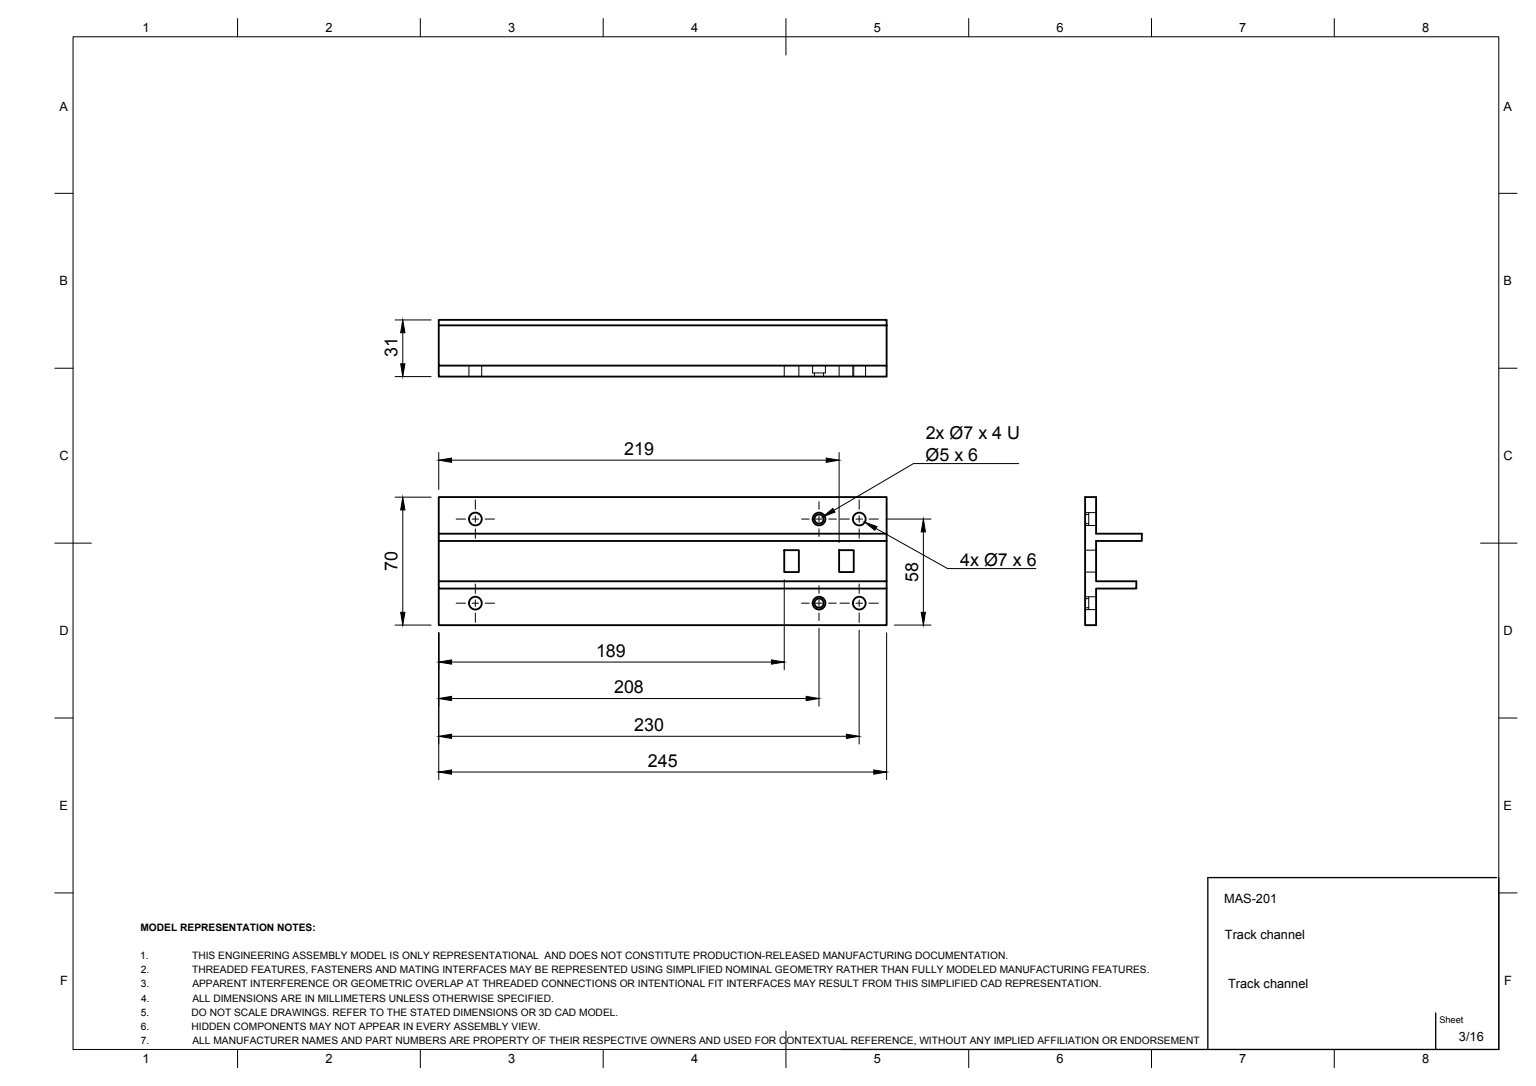
ISO-10303-21;
HEADER;
/* Generated by software containing ST-Developer
 * from STEP Tools, Inc. (www.steptools.com) 
 */

FILE_DESCRIPTION(
/* description */ ('Independent manual two-gate roller-track escapement for nominal30mm d
iameter20mm wide feed rollers. Opposed gates are driven by native capt
ured pin-slot loops with positive curved-slot travel stops at\X\B116de
g. Repeated gate/pin/washer/clip instances, adapted native common bear
ing families, full retaining lips and rotating polymer grip. External 
workpieces, gravity feeder/incline and mount anchors outside assembly.
 No powered-feed compatibility, impact, capacity, safety, force, wear 
or life rating.'),
/* implementation_level */ '2;1');

FILE_NAME(
/* name */ 'Track channel.step',
/* time_stamp */ '2026-11-08T18:43:23-08:00',
/* author */ (''),
/* organization */ (''),
/* preprocessor_version */ 'ST-DEVELOPER v20.2',
/* originating_system */ 'Autodesk Translation Framework v15.17.0.0',
/* authorisation */ '');

FILE_SCHEMA (('AUTOMOTIVE_DESIGN { 1 0 10303 214 3 1 1 }'));
ENDSEC;

DATA;
#10=MECHANICAL_DESIGN_GEOMETRIC_PRESENTATION_REPRESENTATION('',(#455),#19863);
#417=SHAPE_REPRESENTATION_RELATIONSHIP('SRR','None',#19935,#436);
#436=ADVANCED_BREP_SHAPE_REPRESENTATION('',(#474),#19844);
#455=STYLED_ITEM('',(#20039),#474);
#474=MANIFOLD_SOLID_BREP('Body1',#6424);
#493=LINE('',#8742,#958);
#494=LINE('',#8745,#959);
#495=LINE('',#8755,#960);
#496=LINE('',#8758,#961);
#497=LINE('',#8764,#962);
#498=LINE('',#8770,#963);
#499=LINE('',#8776,#964);
#500=LINE('',#8782,#965);
#501=LINE('',#8787,#966);
#502=LINE('',#8789,#967);
#503=LINE('',#8791,#968);
#504=LINE('',#8792,#969);
#505=LINE('',#8795,#970);
#506=LINE('',#8797,#971);
#507=LINE('',#8798,#972);
#508=LINE('',#8801,#973);
#509=LINE('',#8803,#974);
#510=LINE('',#8804,#975);
#511=LINE('',#8806,#976);
#512=LINE('',#8807,#977);
#513=LINE('',#8811,#978);
#514=LINE('',#8813,#979);
#515=LINE('',#8815,#980);
#516=LINE('',#8816,#981);
#517=LINE('',#8819,#982);
#518=LINE('',#8821,#983);
#519=LINE('',#8822,#984);
#520=LINE('',#8825,#985);
#521=LINE('',#8827,#986);
#522=LINE('',#8828,#987);
#523=LINE('',#8830,#988);
#524=LINE('',#8831,#989);
#525=LINE('',#8835,#990);
#526=LINE('',#8837,#991);
#527=LINE('',#8839,#992);
#528=LINE('',#8840,#993);
#529=LINE('',#8844,#994);
#530=LINE('',#8846,#995);
#531=LINE('',#8848,#996);
#532=LINE('',#8849,#997);
#533=LINE('',#8851,#998);
#534=LINE('',#8852,#999);
#535=LINE('',#8855,#1000);
#536=LINE('',#8857,#1001);
#537=LINE('',#8858,#1002);
#538=LINE('',#8861,#1003);
#539=LINE('',#8863,#1004);
#540=LINE('',#8864,#1005);
#541=LINE('',#8867,#1006);
#542=LINE('',#8869,#1007);
#543=LINE('',#8870,#1008);
#544=LINE('',#8874,#1009);
#545=LINE('',#8876,#1010);
#546=LINE('',#8878,#1011);
#547=LINE('',#8879,#1012);
#548=LINE('',#8881,#1013);
#549=LINE('',#8882,#1014);
#550=LINE('',#8885,#1015);
#551=LINE('',#8887,#1016);
#552=LINE('',#8888,#1017);
#553=LINE('',#8892,#1018);
#554=LINE('',#8893,#1019);
#555=LINE('',#8894,#1020);
#556=LINE('',#8897,#1021);
#557=LINE('',#8898,#1022);
#558=LINE('',#8901,#1023);
#559=LINE('',#8902,#1024);
#560=LINE('',#8904,#1025);
#958=VECTOR('',#7205,3.5);
#959=VECTOR('',#7208,2.5);
#960=VECTOR('',#7221,3.5);
#961=VECTOR('',#7224,2.5);
#962=VECTOR('',#7231,3.5);
#963=VECTOR('',#7238,3.5);
#964=VECTOR('',#7245,3.5);
#965=VECTOR('',#7252,3.5);
#966=VECTOR('',#7257,10.);
#967=VECTOR('',#7258,10.);
#968=VECTOR('',#7259,10.);
#969=VECTOR('',#7260,10.);
#970=VECTOR('',#7263,10.);
#971=VECTOR('',#7264,10.);
#972=VECTOR('',#7265,10.);
#973=VECTOR('',#7268,10.);
#974=VECTOR('',#7269,10.);
#975=VECTOR('',#7270,10.);
#976=VECTOR('',#7273,10.);
#977=VECTOR('',#7274,10.);
#978=VECTOR('',#7277,10.);
#979=VECTOR('',#7278,10.);
#980=VECTOR('',#7279,10.);
#981=VECTOR('',#7280,10.);
#982=VECTOR('',#7283,10.);
#983=VECTOR('',#7284,10.);
#984=VECTOR('',#7285,10.);
#985=VECTOR('',#7288,10.);
#986=VECTOR('',#7289,10.);
#987=VECTOR('',#7290,10.);
#988=VECTOR('',#7293,10.);
#989=VECTOR('',#7294,10.);
#990=VECTOR('',#7297,10.);
#991=VECTOR('',#7298,10.);
#992=VECTOR('',#7299,10.);
#993=VECTOR('',#7300,10.);
#994=VECTOR('',#7303,10.);
#995=VECTOR('',#7304,10.);
#996=VECTOR('',#7305,10.);
#997=VECTOR('',#7306,10.);
#998=VECTOR('',#7309,10.);
#999=VECTOR('',#7310,10.);
#1000=VECTOR('',#7313,10.);
#1001=VECTOR('',#7314,10.);
#1002=VECTOR('',#7315,10.);
#1003=VECTOR('',#7318,10.);
#1004=VECTOR('',#7319,10.);
#1005=VECTOR('',#7320,10.);
#1006=VECTOR('',#7323,10.);
#1007=VECTOR('',#7324,10.);
#1008=VECTOR('',#7325,10.);
#1009=VECTOR('',#7328,10.);
#1010=VECTOR('',#7329,10.);
#1011=VECTOR('',#7330,10.);
#1012=VECTOR('',#7331,10.);
#1013=VECTOR('',#7334,10.);
#1014=VECTOR('',#7335,10.);
#1015=VECTOR('',#7338,10.);
#1016=VECTOR('',#7339,10.);
#1017=VECTOR('',#7340,10.);
#1018=VECTOR('',#7343,10.);
#1019=VECTOR('',#7344,10.);
#1020=VECTOR('',#7345,10.);
#1021=VECTOR('',#7348,10.);
#1022=VECTOR('',#7349,10.);
#1023=VECTOR('',#7352,10.);
#1024=VECTOR('',#7353,10.);
#1025=VECTOR('',#7356,10.);
#1423=CYLINDRICAL_SURFACE('',#6658,3.5);
#1424=CYLINDRICAL_SURFACE('',#6660,2.5);
#1425=CYLINDRICAL_SURFACE('',#6665,3.5);
#1426=CYLINDRICAL_SURFACE('',#6667,2.5);
#1427=CYLINDRICAL_SURFACE('',#6669,3.5);
#1428=CYLINDRICAL_SURFACE('',#6672,3.5);
#1429=CYLINDRICAL_SURFACE('',#6675,3.5);
#1430=CYLINDRICAL_SURFACE('',#6678,3.5);
#1616=FACE_BOUND('',#2046,.T.);
#1617=FACE_BOUND('',#2050,.T.);
#1618=FACE_BOUND('',#2069,.T.);
#1619=FACE_BOUND('',#2070,.T.);
#1620=FACE_BOUND('',#2071,.T.);
#1621=FACE_BOUND('',#2073,.T.);
#1622=FACE_BOUND('',#2074,.T.);
#1623=FACE_BOUND('',#2079,.T.);
#1624=FACE_BOUND('',#2080,.T.);
#1625=FACE_BOUND('',#2081,.T.);
#1626=FACE_BOUND('',#2087,.T.);
#1627=FACE_BOUND('',#2088,.T.);
#1628=FACE_BOUND('',#2089,.T.);
#1629=FACE_BOUND('',#2090,.T.);
#1630=FACE_BOUND('',#2091,.T.);
#1631=FACE_BOUND('',#2092,.T.);
#1632=FACE_BOUND('',#2093,.T.);
#1633=FACE_BOUND('',#2094,.T.);
#1687=FACE_OUTER_BOUND('',#2045,.T.);
#1688=FACE_OUTER_BOUND('',#2047,.T.);
#1689=FACE_OUTER_BOUND('',#2048,.T.);
#1690=FACE_OUTER_BOUND('',#2049,.T.);
#1691=FACE_OUTER_BOUND('',#2051,.T.);
#1692=FACE_OUTER_BOUND('',#2052,.T.);
#1693=FACE_OUTER_BOUND('',#2053,.T.);
#1694=FACE_OUTER_BOUND('',#2054,.T.);
#1695=FACE_OUTER_BOUND('',#2055,.T.);
#1696=FACE_OUTER_BOUND('',#2056,.T.);
#1697=FACE_OUTER_BOUND('',#2057,.T.);
#1698=FACE_OUTER_BOUND('',#2058,.T.);
#1699=FACE_OUTER_BOUND('',#2059,.T.);
#1700=FACE_OUTER_BOUND('',#2060,.T.);
#1701=FACE_OUTER_BOUND('',#2061,.T.);
#1702=FACE_OUTER_BOUND('',#2062,.T.);
#1703=FACE_OUTER_BOUND('',#2063,.T.);
#1704=FACE_OUTER_BOUND('',#2064,.T.);
#1705=FACE_OUTER_BOUND('',#2065,.T.);
#1706=FACE_OUTER_BOUND('',#2066,.T.);
#1707=FACE_OUTER_BOUND('',#2067,.T.);
#1708=FACE_OUTER_BOUND('',#2068,.T.);
#1709=FACE_OUTER_BOUND('',#2072,.T.);
#1710=FACE_OUTER_BOUND('',#2075,.T.);
#1711=FACE_OUTER_BOUND('',#2076,.T.);
#1712=FACE_OUTER_BOUND('',#2077,.T.);
#1713=FACE_OUTER_BOUND('',#2078,.T.);
#1714=FACE_OUTER_BOUND('',#2082,.T.);
#1715=FACE_OUTER_BOUND('',#2083,.T.);
#1716=FACE_OUTER_BOUND('',#2084,.T.);
#1717=FACE_OUTER_BOUND('',#2085,.T.);
#1718=FACE_OUTER_BOUND('',#2086,.T.);
#2045=EDGE_LOOP('',(#4115));
#2046=EDGE_LOOP('',(#4116));
#2047=EDGE_LOOP('',(#4117,#4118,#4119,#4120));
#2048=EDGE_LOOP('',(#4121,#4122,#4123,#4124));
#2049=EDGE_LOOP('',(#4125));
#2050=EDGE_LOOP('',(#4126));
#2051=EDGE_LOOP('',(#4127,#4128,#4129,#4130));
#2052=EDGE_LOOP('',(#4131,#4132,#4133,#4134));
#2053=EDGE_LOOP('',(#4135,#4136,#4137,#4138));
#2054=EDGE_LOOP('',(#4139,#4140,#4141,#4142));
#2055=EDGE_LOOP('',(#4143,#4144,#4145,#4146));
#2056=EDGE_LOOP('',(#4147,#4148,#4149,#4150));
#2057=EDGE_LOOP('',(#4151,#4152,#4153,#4154));
#2058=EDGE_LOOP('',(#4155,#4156,#4157,#4158));
#2059=EDGE_LOOP('',(#4159,#4160,#4161,#4162));
#2060=EDGE_LOOP('',(#4163,#4164,#4165,#4166));
#2061=EDGE_LOOP('',(#4167,#4168,#4169,#4170));
#2062=EDGE_LOOP('',(#4171,#4172,#4173,#4174));
#2063=EDGE_LOOP('',(#4175,#4176,#4177,#4178));
#2064=EDGE_LOOP('',(#4179,#4180,#4181,#4182));
#2065=EDGE_LOOP('',(#4183,#4184,#4185,#4186));
#2066=EDGE_LOOP('',(#4187,#4188,#4189,#4190));
#2067=EDGE_LOOP('',(#4191,#4192,#4193,#4194));
#2068=EDGE_LOOP('',(#4195,#4196,#4197,#4198));
#2069=EDGE_LOOP('',(#4199));
#2070=EDGE_LOOP('',(#4200));
#2071=EDGE_LOOP('',(#4201));
#2072=EDGE_LOOP('',(#4202,#4203,#4204,#4205));
#2073=EDGE_LOOP('',(#4206,#4207,#4208,#4209));
#2074=EDGE_LOOP('',(#4210,#4211,#4212,#4213));
#2075=EDGE_LOOP('',(#4214,#4215,#4216,#4217));
#2076=EDGE_LOOP('',(#4218,#4219,#4220,#4221));
#2077=EDGE_LOOP('',(#4222,#4223,#4224,#4225));
#2078=EDGE_LOOP('',(#4226,#4227,#4228,#4229));
#2079=EDGE_LOOP('',(#4230));
#2080=EDGE_LOOP('',(#4231));
#2081=EDGE_LOOP('',(#4232));
#2082=EDGE_LOOP('',(#4233,#4234,#4235,#4236));
#2083=EDGE_LOOP('',(#4237,#4238,#4239,#4240,#4241,#4242,#4243,#4244,#4245,
#4246,#4247,#4248));
#2084=EDGE_LOOP('',(#4249,#4250,#4251,#4252));
#2085=EDGE_LOOP('',(#4253,#4254,#4255,#4256,#4257,#4258,#4259,#4260,#4261,
#4262,#4263,#4264));
#2086=EDGE_LOOP('',(#4265,#4266,#4267,#4268));
#2087=EDGE_LOOP('',(#4269));
#2088=EDGE_LOOP('',(#4270));
#2089=EDGE_LOOP('',(#4271));
#2090=EDGE_LOOP('',(#4272));
#2091=EDGE_LOOP('',(#4273,#4274,#4275,#4276));
#2092=EDGE_LOOP('',(#4277,#4278,#4279,#4280));
#2093=EDGE_LOOP('',(#4281));
#2094=EDGE_LOOP('',(#4282));
#2474=CIRCLE('',#6656,3.5);
#2475=CIRCLE('',#6657,2.5);
#2476=CIRCLE('',#6659,3.5);
#2477=CIRCLE('',#6661,2.5);
#2478=CIRCLE('',#6663,3.5);
#2479=CIRCLE('',#6664,2.5);
#2480=CIRCLE('',#6666,3.5);
#2481=CIRCLE('',#6668,2.5);
#2482=CIRCLE('',#6670,3.5);
#2483=CIRCLE('',#6671,3.5);
#2484=CIRCLE('',#6673,3.5);
#2485=CIRCLE('',#6674,3.5);
#2486=CIRCLE('',#6676,3.5);
#2487=CIRCLE('',#6677,3.5);
#2488=CIRCLE('',#6679,3.5);
#2489=CIRCLE('',#6680,3.5);
#2618=VERTEX_POINT('',#8735);
#2619=VERTEX_POINT('',#8737);
#2620=VERTEX_POINT('',#8740);
#2621=VERTEX_POINT('',#8744);
#2622=VERTEX_POINT('',#8748);
#2623=VERTEX_POINT('',#8750);
#2624=VERTEX_POINT('',#8753);
#2625=VERTEX_POINT('',#8757);
#2626=VERTEX_POINT('',#8761);
#2627=VERTEX_POINT('',#8763);
#2628=VERTEX_POINT('',#8767);
#2629=VERTEX_POINT('',#8769);
#2630=VERTEX_POINT('',#8773);
#2631=VERTEX_POINT('',#8775);
#2632=VERTEX_POINT('',#8779);
#2633=VERTEX_POINT('',#8781);
#2634=VERTEX_POINT('',#8785);
#2635=VERTEX_POINT('',#8786);
#2636=VERTEX_POINT('',#8788);
#2637=VERTEX_POINT('',#8790);
#2638=VERTEX_POINT('',#8794);
#2639=VERTEX_POINT('',#8796);
#2640=VERTEX_POINT('',#8800);
#2641=VERTEX_POINT('',#8802);
#2642=VERTEX_POINT('',#8809);
#2643=VERTEX_POINT('',#8810);
#2644=VERTEX_POINT('',#8812);
#2645=VERTEX_POINT('',#8814);
#2646=VERTEX_POINT('',#8818);
#2647=VERTEX_POINT('',#8820);
#2648=VERTEX_POINT('',#8824);
#2649=VERTEX_POINT('',#8826);
#2650=VERTEX_POINT('',#8833);
#2651=VERTEX_POINT('',#8834);
#2652=VERTEX_POINT('',#8836);
#2653=VERTEX_POINT('',#8838);
#2654=VERTEX_POINT('',#8842);
#2655=VERTEX_POINT('',#8843);
#2656=VERTEX_POINT('',#8845);
#2657=VERTEX_POINT('',#8847);
#2658=VERTEX_POINT('',#8854);
#2659=VERTEX_POINT('',#8856);
#2660=VERTEX_POINT('',#8860);
#2661=VERTEX_POINT('',#8862);
#2662=VERTEX_POINT('',#8866);
#2663=VERTEX_POINT('',#8868);
#2664=VERTEX_POINT('',#8872);
#2665=VERTEX_POINT('',#8873);
#2666=VERTEX_POINT('',#8875);
#2667=VERTEX_POINT('',#8877);
#2668=VERTEX_POINT('',#8884);
#2669=VERTEX_POINT('',#8886);
#2670=VERTEX_POINT('',#8890);
#2671=VERTEX_POINT('',#8891);
#2672=VERTEX_POINT('',#8896);
#2673=VERTEX_POINT('',#8900);
#3216=EDGE_CURVE('',#2618,#2618,#2474,.T.);
#3217=EDGE_CURVE('',#2619,#2619,#2475,.T.);
#3218=EDGE_CURVE('',#2620,#2620,#2476,.T.);
#3219=EDGE_CURVE('',#2620,#2618,#493,.T.);
#3220=EDGE_CURVE('',#2619,#2621,#494,.T.);
#3221=EDGE_CURVE('',#2621,#2621,#2477,.T.);
#3222=EDGE_CURVE('',#2622,#2622,#2478,.T.);
#3223=EDGE_CURVE('',#2623,#2623,#2479,.T.);
#3224=EDGE_CURVE('',#2624,#2624,#2480,.T.);
#3225=EDGE_CURVE('',#2624,#2622,#495,.T.);
#3226=EDGE_CURVE('',#2623,#2625,#496,.T.);
#3227=EDGE_CURVE('',#2625,#2625,#2481,.T.);
#3228=EDGE_CURVE('',#2626,#2626,#2482,.T.);
#3229=EDGE_CURVE('',#2626,#2627,#497,.T.);
#3230=EDGE_CURVE('',#2627,#2627,#2483,.T.);
#3231=EDGE_CURVE('',#2628,#2628,#2484,.T.);
#3232=EDGE_CURVE('',#2628,#2629,#498,.T.);
#3233=EDGE_CURVE('',#2629,#2629,#2485,.T.);
#3234=EDGE_CURVE('',#2630,#2630,#2486,.T.);
#3235=EDGE_CURVE('',#2630,#2631,#499,.T.);
#3236=EDGE_CURVE('',#2631,#2631,#2487,.T.);
#3237=EDGE_CURVE('',#2632,#2632,#2488,.T.);
#3238=EDGE_CURVE('',#2632,#2633,#500,.T.);
#3239=EDGE_CURVE('',#2633,#2633,#2489,.T.);
#3240=EDGE_CURVE('',#2634,#2635,#501,.T.);
#3241=EDGE_CURVE('',#2634,#2636,#502,.T.);
#3242=EDGE_CURVE('',#2637,#2636,#503,.T.);
#3243=EDGE_CURVE('',#2635,#2637,#504,.T.);
#3244=EDGE_CURVE('',#2638,#2634,#505,.T.);
#3245=EDGE_CURVE('',#2638,#2639,#506,.T.);
#3246=EDGE_CURVE('',#2636,#2639,#507,.T.);
#3247=EDGE_CURVE('',#2640,#2638,#508,.T.);
#3248=EDGE_CURVE('',#2640,#2641,#509,.T.);
#3249=EDGE_CURVE('',#2639,#2641,#510,.T.);
#3250=EDGE_CURVE('',#2635,#2640,#511,.T.);
#3251=EDGE_CURVE('',#2641,#2637,#512,.T.);
#3252=EDGE_CURVE('',#2642,#2643,#513,.T.);
#3253=EDGE_CURVE('',#2642,#2644,#514,.T.);
#3254=EDGE_CURVE('',#2645,#2644,#515,.T.);
#3255=EDGE_CURVE('',#2643,#2645,#516,.T.);
#3256=EDGE_CURVE('',#2646,#2642,#517,.T.);
#3257=EDGE_CURVE('',#2646,#2647,#518,.T.);
#3258=EDGE_CURVE('',#2644,#2647,#519,.T.);
#3259=EDGE_CURVE('',#2648,#2646,#520,.T.);
#3260=EDGE_CURVE('',#2648,#2649,#521,.T.);
#3261=EDGE_CURVE('',#2647,#2649,#522,.T.);
#3262=EDGE_CURVE('',#2643,#2648,#523,.T.);
#3263=EDGE_CURVE('',#2649,#2645,#524,.T.);
#3264=EDGE_CURVE('',#2650,#2651,#525,.T.);
#3265=EDGE_CURVE('',#2650,#2652,#526,.F.);
#3266=EDGE_CURVE('',#2653,#2652,#527,.T.);
#3267=EDGE_CURVE('',#2651,#2653,#528,.T.);
#3268=EDGE_CURVE('',#2654,#2655,#529,.T.);
#3269=EDGE_CURVE('',#2654,#2656,#530,.T.);
#3270=EDGE_CURVE('',#2657,#2656,#531,.T.);
#3271=EDGE_CURVE('',#2655,#2657,#532,.T.);
#3272=EDGE_CURVE('',#2652,#2657,#533,.F.);
#3273=EDGE_CURVE('',#2656,#2653,#534,.T.);
#3274=EDGE_CURVE('',#2651,#2658,#535,.T.);
#3275=EDGE_CURVE('',#2658,#2659,#536,.F.);
#3276=EDGE_CURVE('',#2659,#2650,#537,.F.);
#3277=EDGE_CURVE('',#2655,#2660,#538,.F.);
#3278=EDGE_CURVE('',#2660,#2661,#539,.T.);
#3279=EDGE_CURVE('',#2661,#2654,#540,.T.);
#3280=EDGE_CURVE('',#2660,#2662,#541,.F.);
#3281=EDGE_CURVE('',#2663,#2662,#542,.T.);
#3282=EDGE_CURVE('',#2661,#2663,#543,.T.);
#3283=EDGE_CURVE('',#2664,#2665,#544,.T.);
#3284=EDGE_CURVE('',#2664,#2666,#545,.T.);
#3285=EDGE_CURVE('',#2667,#2666,#546,.T.);
#3286=EDGE_CURVE('',#2665,#2667,#547,.T.);
#3287=EDGE_CURVE('',#2662,#2667,#548,.F.);
#3288=EDGE_CURVE('',#2666,#2663,#549,.T.);
#3289=EDGE_CURVE('',#2665,#2668,#550,.F.);
#3290=EDGE_CURVE('',#2668,#2669,#551,.F.);
#3291=EDGE_CURVE('',#2669,#2664,#552,.T.);
#3292=EDGE_CURVE('',#2670,#2671,#553,.F.);
#3293=EDGE_CURVE('',#2671,#2659,#554,.F.);
#3294=EDGE_CURVE('',#2670,#2658,#555,.F.);
#3295=EDGE_CURVE('',#2672,#2670,#556,.T.);
#3296=EDGE_CURVE('',#2672,#2669,#557,.T.);
#3297=EDGE_CURVE('',#2673,#2672,#558,.F.);
#3298=EDGE_CURVE('',#2673,#2668,#559,.T.);
#3299=EDGE_CURVE('',#2671,#2673,#560,.F.);
#4115=ORIENTED_EDGE('',*,*,#3216,.F.);
#4116=ORIENTED_EDGE('',*,*,#3217,.T.);
#4117=ORIENTED_EDGE('',*,*,#3218,.F.);
#4118=ORIENTED_EDGE('',*,*,#3219,.T.);
#4119=ORIENTED_EDGE('',*,*,#3216,.T.);
#4120=ORIENTED_EDGE('',*,*,#3219,.F.);
#4121=ORIENTED_EDGE('',*,*,#3217,.F.);
#4122=ORIENTED_EDGE('',*,*,#3220,.T.);
#4123=ORIENTED_EDGE('',*,*,#3221,.F.);
#4124=ORIENTED_EDGE('',*,*,#3220,.F.);
#4125=ORIENTED_EDGE('',*,*,#3222,.F.);
#4126=ORIENTED_EDGE('',*,*,#3223,.T.);
#4127=ORIENTED_EDGE('',*,*,#3224,.F.);
#4128=ORIENTED_EDGE('',*,*,#3225,.T.);
#4129=ORIENTED_EDGE('',*,*,#3222,.T.);
#4130=ORIENTED_EDGE('',*,*,#3225,.F.);
#4131=ORIENTED_EDGE('',*,*,#3223,.F.);
#4132=ORIENTED_EDGE('',*,*,#3226,.T.);
#4133=ORIENTED_EDGE('',*,*,#3227,.F.);
#4134=ORIENTED_EDGE('',*,*,#3226,.F.);
#4135=ORIENTED_EDGE('',*,*,#3228,.F.);
#4136=ORIENTED_EDGE('',*,*,#3229,.T.);
#4137=ORIENTED_EDGE('',*,*,#3230,.F.);
#4138=ORIENTED_EDGE('',*,*,#3229,.F.);
#4139=ORIENTED_EDGE('',*,*,#3231,.F.);
#4140=ORIENTED_EDGE('',*,*,#3232,.T.);
#4141=ORIENTED_EDGE('',*,*,#3233,.F.);
#4142=ORIENTED_EDGE('',*,*,#3232,.F.);
#4143=ORIENTED_EDGE('',*,*,#3234,.F.);
#4144=ORIENTED_EDGE('',*,*,#3235,.T.);
#4145=ORIENTED_EDGE('',*,*,#3236,.F.);
#4146=ORIENTED_EDGE('',*,*,#3235,.F.);
#4147=ORIENTED_EDGE('',*,*,#3237,.F.);
#4148=ORIENTED_EDGE('',*,*,#3238,.T.);
#4149=ORIENTED_EDGE('',*,*,#3239,.F.);
#4150=ORIENTED_EDGE('',*,*,#3238,.F.);
#4151=ORIENTED_EDGE('',*,*,#3240,.F.);
#4152=ORIENTED_EDGE('',*,*,#3241,.T.);
#4153=ORIENTED_EDGE('',*,*,#3242,.F.);
#4154=ORIENTED_EDGE('',*,*,#3243,.F.);
#4155=ORIENTED_EDGE('',*,*,#3244,.F.);
#4156=ORIENTED_EDGE('',*,*,#3245,.T.);
#4157=ORIENTED_EDGE('',*,*,#3246,.F.);
#4158=ORIENTED_EDGE('',*,*,#3241,.F.);
#4159=ORIENTED_EDGE('',*,*,#3247,.F.);
#4160=ORIENTED_EDGE('',*,*,#3248,.T.);
#4161=ORIENTED_EDGE('',*,*,#3249,.F.);
#4162=ORIENTED_EDGE('',*,*,#3245,.F.);
#4163=ORIENTED_EDGE('',*,*,#3250,.F.);
#4164=ORIENTED_EDGE('',*,*,#3243,.T.);
#4165=ORIENTED_EDGE('',*,*,#3251,.F.);
#4166=ORIENTED_EDGE('',*,*,#3248,.F.);
#4167=ORIENTED_EDGE('',*,*,#3252,.F.);
#4168=ORIENTED_EDGE('',*,*,#3253,.T.);
#4169=ORIENTED_EDGE('',*,*,#3254,.F.);
#4170=ORIENTED_EDGE('',*,*,#3255,.F.);
#4171=ORIENTED_EDGE('',*,*,#3256,.F.);
#4172=ORIENTED_EDGE('',*,*,#3257,.T.);
#4173=ORIENTED_EDGE('',*,*,#3258,.F.);
#4174=ORIENTED_EDGE('',*,*,#3253,.F.);
#4175=ORIENTED_EDGE('',*,*,#3259,.F.);
#4176=ORIENTED_EDGE('',*,*,#3260,.T.);
#4177=ORIENTED_EDGE('',*,*,#3261,.F.);
#4178=ORIENTED_EDGE('',*,*,#3257,.F.);
#4179=ORIENTED_EDGE('',*,*,#3262,.F.);
#4180=ORIENTED_EDGE('',*,*,#3255,.T.);
#4181=ORIENTED_EDGE('',*,*,#3263,.F.);
#4182=ORIENTED_EDGE('',*,*,#3260,.F.);
#4183=ORIENTED_EDGE('',*,*,#3264,.F.);
#4184=ORIENTED_EDGE('',*,*,#3265,.T.);
#4185=ORIENTED_EDGE('',*,*,#3266,.F.);
#4186=ORIENTED_EDGE('',*,*,#3267,.F.);
#4187=ORIENTED_EDGE('',*,*,#3268,.F.);
#4188=ORIENTED_EDGE('',*,*,#3269,.T.);
#4189=ORIENTED_EDGE('',*,*,#3270,.F.);
#4190=ORIENTED_EDGE('',*,*,#3271,.F.);
#4191=ORIENTED_EDGE('',*,*,#3272,.T.);
#4192=ORIENTED_EDGE('',*,*,#3270,.T.);
#4193=ORIENTED_EDGE('',*,*,#3273,.T.);
#4194=ORIENTED_EDGE('',*,*,#3266,.T.);
#4195=ORIENTED_EDGE('',*,*,#3264,.T.);
#4196=ORIENTED_EDGE('',*,*,#3274,.T.);
#4197=ORIENTED_EDGE('',*,*,#3275,.T.);
#4198=ORIENTED_EDGE('',*,*,#3276,.T.);
#4199=ORIENTED_EDGE('',*,*,#3224,.T.);
#4200=ORIENTED_EDGE('',*,*,#3234,.T.);
#4201=ORIENTED_EDGE('',*,*,#3237,.T.);
#4202=ORIENTED_EDGE('',*,*,#3268,.T.);
#4203=ORIENTED_EDGE('',*,*,#3277,.T.);
#4204=ORIENTED_EDGE('',*,*,#3278,.T.);
#4205=ORIENTED_EDGE('',*,*,#3279,.T.);
#4206=ORIENTED_EDGE('',*,*,#3240,.T.);
#4207=ORIENTED_EDGE('',*,*,#3250,.T.);
#4208=ORIENTED_EDGE('',*,*,#3247,.T.);
#4209=ORIENTED_EDGE('',*,*,#3244,.T.);
#4210=ORIENTED_EDGE('',*,*,#3252,.T.);
#4211=ORIENTED_EDGE('',*,*,#3262,.T.);
#4212=ORIENTED_EDGE('',*,*,#3259,.T.);
#4213=ORIENTED_EDGE('',*,*,#3256,.T.);
#4214=ORIENTED_EDGE('',*,*,#3278,.F.);
#4215=ORIENTED_EDGE('',*,*,#3280,.T.);
#4216=ORIENTED_EDGE('',*,*,#3281,.F.);
#4217=ORIENTED_EDGE('',*,*,#3282,.F.);
#4218=ORIENTED_EDGE('',*,*,#3283,.F.);
#4219=ORIENTED_EDGE('',*,*,#3284,.T.);
#4220=ORIENTED_EDGE('',*,*,#3285,.F.);
#4221=ORIENTED_EDGE('',*,*,#3286,.F.);
#4222=ORIENTED_EDGE('',*,*,#3287,.T.);
#4223=ORIENTED_EDGE('',*,*,#3285,.T.);
#4224=ORIENTED_EDGE('',*,*,#3288,.T.);
#4225=ORIENTED_EDGE('',*,*,#3281,.T.);
#4226=ORIENTED_EDGE('',*,*,#3283,.T.);
#4227=ORIENTED_EDGE('',*,*,#3289,.T.);
#4228=ORIENTED_EDGE('',*,*,#3290,.T.);
#4229=ORIENTED_EDGE('',*,*,#3291,.T.);
#4230=ORIENTED_EDGE('',*,*,#3218,.T.);
#4231=ORIENTED_EDGE('',*,*,#3228,.T.);
#4232=ORIENTED_EDGE('',*,*,#3231,.T.);
#4233=ORIENTED_EDGE('',*,*,#3292,.T.);
#4234=ORIENTED_EDGE('',*,*,#3293,.T.);
#4235=ORIENTED_EDGE('',*,*,#3275,.F.);
#4236=ORIENTED_EDGE('',*,*,#3294,.F.);
#4237=ORIENTED_EDGE('',*,*,#3295,.T.);
#4238=ORIENTED_EDGE('',*,*,#3294,.T.);
#4239=ORIENTED_EDGE('',*,*,#3274,.F.);
#4240=ORIENTED_EDGE('',*,*,#3267,.T.);
#4241=ORIENTED_EDGE('',*,*,#3273,.F.);
#4242=ORIENTED_EDGE('',*,*,#3269,.F.);
#4243=ORIENTED_EDGE('',*,*,#3279,.F.);
#4244=ORIENTED_EDGE('',*,*,#3282,.T.);
#4245=ORIENTED_EDGE('',*,*,#3288,.F.);
#4246=ORIENTED_EDGE('',*,*,#3284,.F.);
#4247=ORIENTED_EDGE('',*,*,#3291,.F.);
#4248=ORIENTED_EDGE('',*,*,#3296,.F.);
#4249=ORIENTED_EDGE('',*,*,#3297,.T.);
#4250=ORIENTED_EDGE('',*,*,#3296,.T.);
#4251=ORIENTED_EDGE('',*,*,#3290,.F.);
#4252=ORIENTED_EDGE('',*,*,#3298,.F.);
#4253=ORIENTED_EDGE('',*,*,#3299,.T.);
#4254=ORIENTED_EDGE('',*,*,#3298,.T.);
#4255=ORIENTED_EDGE('',*,*,#3289,.F.);
#4256=ORIENTED_EDGE('',*,*,#3286,.T.);
#4257=ORIENTED_EDGE('',*,*,#3287,.F.);
#4258=ORIENTED_EDGE('',*,*,#3280,.F.);
#4259=ORIENTED_EDGE('',*,*,#3277,.F.);
#4260=ORIENTED_EDGE('',*,*,#3271,.T.);
#4261=ORIENTED_EDGE('',*,*,#3272,.F.);
#4262=ORIENTED_EDGE('',*,*,#3265,.F.);
#4263=ORIENTED_EDGE('',*,*,#3276,.F.);
#4264=ORIENTED_EDGE('',*,*,#3293,.F.);
#4265=ORIENTED_EDGE('',*,*,#3299,.F.);
#4266=ORIENTED_EDGE('',*,*,#3292,.F.);
#4267=ORIENTED_EDGE('',*,*,#3295,.F.);
#4268=ORIENTED_EDGE('',*,*,#3297,.F.);
#4269=ORIENTED_EDGE('',*,*,#3230,.T.);
#4270=ORIENTED_EDGE('',*,*,#3233,.T.);
#4271=ORIENTED_EDGE('',*,*,#3236,.T.);
#4272=ORIENTED_EDGE('',*,*,#3239,.T.);
#4273=ORIENTED_EDGE('',*,*,#3242,.T.);
#4274=ORIENTED_EDGE('',*,*,#3246,.T.);
#4275=ORIENTED_EDGE('',*,*,#3249,.T.);
#4276=ORIENTED_EDGE('',*,*,#3251,.T.);
#4277=ORIENTED_EDGE('',*,*,#3254,.T.);
#4278=ORIENTED_EDGE('',*,*,#3258,.T.);
#4279=ORIENTED_EDGE('',*,*,#3261,.T.);
#4280=ORIENTED_EDGE('',*,*,#3263,.T.);
#4281=ORIENTED_EDGE('',*,*,#3227,.T.);
#4282=ORIENTED_EDGE('',*,*,#3221,.T.);
#5913=PLANE('',#6655);
#5914=PLANE('',#6662);
#5915=PLANE('',#6681);
#5916=PLANE('',#6682);
#5917=PLANE('',#6683);
#5918=PLANE('',#6684);
#5919=PLANE('',#6685);
#5920=PLANE('',#6686);
#5921=PLANE('',#6687);
#5922=PLANE('',#6688);
#5923=PLANE('',#6689);
#5924=PLANE('',#6690);
#5925=PLANE('',#6691);
#5926=PLANE('',#6692);
#5927=PLANE('',#6693);
#5928=PLANE('',#6694);
#5929=PLANE('',#6695);
#5930=PLANE('',#6696);
#5931=PLANE('',#6697);
#5932=PLANE('',#6698);
#5933=PLANE('',#6699);
#5934=PLANE('',#6700);
#5935=PLANE('',#6701);
#5936=PLANE('',#6702);
#6066=ADVANCED_FACE('',(#1687,#1616),#5913,.F.);
#6067=ADVANCED_FACE('',(#1688),#1423,.F.);
#6068=ADVANCED_FACE('',(#1689),#1424,.F.);
#6069=ADVANCED_FACE('',(#1690,#1617),#5914,.F.);
#6070=ADVANCED_FACE('',(#1691),#1425,.F.);
#6071=ADVANCED_FACE('',(#1692),#1426,.F.);
#6072=ADVANCED_FACE('',(#1693),#1427,.F.);
#6073=ADVANCED_FACE('',(#1694),#1428,.F.);
#6074=ADVANCED_FACE('',(#1695),#1429,.F.);
#6075=ADVANCED_FACE('',(#1696),#1430,.F.);
#6076=ADVANCED_FACE('',(#1697),#5915,.F.);
#6077=ADVANCED_FACE('',(#1698),#5916,.F.);
#6078=ADVANCED_FACE('',(#1699),#5917,.F.);
#6079=ADVANCED_FACE('',(#1700),#5918,.F.);
#6080=ADVANCED_FACE('',(#1701),#5919,.F.);
#6081=ADVANCED_FACE('',(#1702),#5920,.F.);
#6082=ADVANCED_FACE('',(#1703),#5921,.F.);
#6083=ADVANCED_FACE('',(#1704),#5922,.F.);
#6084=ADVANCED_FACE('',(#1705),#5923,.T.);
#6085=ADVANCED_FACE('',(#1706),#5924,.T.);
#6086=ADVANCED_FACE('',(#1707),#5925,.T.);
#6087=ADVANCED_FACE('',(#1708,#1618,#1619,#1620),#5926,.T.);
#6088=ADVANCED_FACE('',(#1709,#1621,#1622),#5927,.T.);
#6089=ADVANCED_FACE('',(#1710),#5928,.T.);
#6090=ADVANCED_FACE('',(#1711),#5929,.T.);
#6091=ADVANCED_FACE('',(#1712),#5930,.T.);
#6092=ADVANCED_FACE('',(#1713,#1623,#1624,#1625),#5931,.T.);
#6093=ADVANCED_FACE('',(#1714),#5932,.T.);
#6094=ADVANCED_FACE('',(#1715),#5933,.T.);
#6095=ADVANCED_FACE('',(#1716),#5934,.T.);
#6096=ADVANCED_FACE('',(#1717),#5935,.T.);
#6097=ADVANCED_FACE('',(#1718,#1626,#1627,#1628,#1629,#1630,#1631,#1632,
#1633),#5936,.F.);
#6424=CLOSED_SHELL('',(#6066,#6067,#6068,#6069,#6070,#6071,#6072,#6073,
#6074,#6075,#6076,#6077,#6078,#6079,#6080,#6081,#6082,#6083,#6084,#6085,
#6086,#6087,#6088,#6089,#6090,#6091,#6092,#6093,#6094,#6095,#6096,#6097));
#6654=AXIS2_PLACEMENT_3D('',#8733,#7193,#7194);
#6655=AXIS2_PLACEMENT_3D('',#8734,#7195,#7196);
#6656=AXIS2_PLACEMENT_3D('',#8736,#7197,#7198);
#6657=AXIS2_PLACEMENT_3D('',#8738,#7199,#7200);
#6658=AXIS2_PLACEMENT_3D('',#8739,#7201,#7202);
#6659=AXIS2_PLACEMENT_3D('',#8741,#7203,#7204);
#6660=AXIS2_PLACEMENT_3D('',#8743,#7206,#7207);
#6661=AXIS2_PLACEMENT_3D('',#8746,#7209,#7210);
#6662=AXIS2_PLACEMENT_3D('',#8747,#7211,#7212);
#6663=AXIS2_PLACEMENT_3D('',#8749,#7213,#7214);
#6664=AXIS2_PLACEMENT_3D('',#8751,#7215,#7216);
#6665=AXIS2_PLACEMENT_3D('',#8752,#7217,#7218);
#6666=AXIS2_PLACEMENT_3D('',#8754,#7219,#7220);
#6667=AXIS2_PLACEMENT_3D('',#8756,#7222,#7223);
#6668=AXIS2_PLACEMENT_3D('',#8759,#7225,#7226);
#6669=AXIS2_PLACEMENT_3D('',#8760,#7227,#7228);
#6670=AXIS2_PLACEMENT_3D('',#8762,#7229,#7230);
#6671=AXIS2_PLACEMENT_3D('',#8765,#7232,#7233);
#6672=AXIS2_PLACEMENT_3D('',#8766,#7234,#7235);
#6673=AXIS2_PLACEMENT_3D('',#8768,#7236,#7237);
#6674=AXIS2_PLACEMENT_3D('',#8771,#7239,#7240);
#6675=AXIS2_PLACEMENT_3D('',#8772,#7241,#7242);
#6676=AXIS2_PLACEMENT_3D('',#8774,#7243,#7244);
#6677=AXIS2_PLACEMENT_3D('',#8777,#7246,#7247);
#6678=AXIS2_PLACEMENT_3D('',#8778,#7248,#7249);
#6679=AXIS2_PLACEMENT_3D('',#8780,#7250,#7251);
#6680=AXIS2_PLACEMENT_3D('',#8783,#7253,#7254);
#6681=AXIS2_PLACEMENT_3D('',#8784,#7255,#7256);
#6682=AXIS2_PLACEMENT_3D('',#8793,#7261,#7262);
#6683=AXIS2_PLACEMENT_3D('',#8799,#7266,#7267);
#6684=AXIS2_PLACEMENT_3D('',#8805,#7271,#7272);
#6685=AXIS2_PLACEMENT_3D('',#8808,#7275,#7276);
#6686=AXIS2_PLACEMENT_3D('',#8817,#7281,#7282);
#6687=AXIS2_PLACEMENT_3D('',#8823,#7286,#7287);
#6688=AXIS2_PLACEMENT_3D('',#8829,#7291,#7292);
#6689=AXIS2_PLACEMENT_3D('',#8832,#7295,#7296);
#6690=AXIS2_PLACEMENT_3D('',#8841,#7301,#7302);
#6691=AXIS2_PLACEMENT_3D('',#8850,#7307,#7308);
#6692=AXIS2_PLACEMENT_3D('',#8853,#7311,#7312);
#6693=AXIS2_PLACEMENT_3D('',#8859,#7316,#7317);
#6694=AXIS2_PLACEMENT_3D('',#8865,#7321,#7322);
#6695=AXIS2_PLACEMENT_3D('',#8871,#7326,#7327);
#6696=AXIS2_PLACEMENT_3D('',#8880,#7332,#7333);
#6697=AXIS2_PLACEMENT_3D('',#8883,#7336,#7337);
#6698=AXIS2_PLACEMENT_3D('',#8889,#7341,#7342);
#6699=AXIS2_PLACEMENT_3D('',#8895,#7346,#7347);
#6700=AXIS2_PLACEMENT_3D('',#8899,#7350,#7351);
#6701=AXIS2_PLACEMENT_3D('',#8903,#7354,#7355);
#6702=AXIS2_PLACEMENT_3D('',#8905,#7357,#7358);
#7193=DIRECTION('axis',(0.,0.,1.));
#7194=DIRECTION('refdir',(1.,0.,0.));
#7195=DIRECTION('center_axis',(0.,0.,-1.));
#7196=DIRECTION('ref_axis',(1.,0.,0.));
#7197=DIRECTION('center_axis',(0.,0.,-1.));
#7198=DIRECTION('ref_axis',(1.,0.,0.));
#7199=DIRECTION('center_axis',(0.,0.,-1.));
#7200=DIRECTION('ref_axis',(1.,0.,0.));
#7201=DIRECTION('center_axis',(0.,0.,-1.));
#7202=DIRECTION('ref_axis',(1.,0.,0.));
#7203=DIRECTION('center_axis',(0.,0.,-1.));
#7204=DIRECTION('ref_axis',(1.,0.,0.));
#7205=DIRECTION('',(0.,0.,-1.));
#7206=DIRECTION('center_axis',(0.,0.,-1.));
#7207=DIRECTION('ref_axis',(1.,0.,0.));
#7208=DIRECTION('',(0.,0.,-1.));
#7209=DIRECTION('center_axis',(0.,0.,1.));
#7210=DIRECTION('ref_axis',(1.,0.,0.));
#7211=DIRECTION('center_axis',(0.,0.,-1.));
#7212=DIRECTION('ref_axis',(1.,0.,0.));
#7213=DIRECTION('center_axis',(0.,0.,-1.));
#7214=DIRECTION('ref_axis',(1.,0.,0.));
#7215=DIRECTION('center_axis',(0.,0.,-1.));
#7216=DIRECTION('ref_axis',(1.,0.,0.));
#7217=DIRECTION('center_axis',(0.,0.,-1.));
#7218=DIRECTION('ref_axis',(1.,0.,0.));
#7219=DIRECTION('center_axis',(0.,0.,-1.));
#7220=DIRECTION('ref_axis',(1.,0.,0.));
#7221=DIRECTION('',(0.,0.,-1.));
#7222=DIRECTION('center_axis',(0.,0.,-1.));
#7223=DIRECTION('ref_axis',(1.,0.,0.));
#7224=DIRECTION('',(0.,0.,-1.));
#7225=DIRECTION('center_axis',(0.,0.,1.));
#7226=DIRECTION('ref_axis',(1.,0.,0.));
#7227=DIRECTION('center_axis',(0.,0.,-1.));
#7228=DIRECTION('ref_axis',(1.,0.,0.));
#7229=DIRECTION('center_axis',(0.,0.,-1.));
#7230=DIRECTION('ref_axis',(1.,0.,0.));
#7231=DIRECTION('',(0.,0.,-1.));
#7232=DIRECTION('center_axis',(0.,0.,1.));
#7233=DIRECTION('ref_axis',(1.,0.,0.));
#7234=DIRECTION('center_axis',(0.,0.,-1.));
#7235=DIRECTION('ref_axis',(1.,0.,0.));
#7236=DIRECTION('center_axis',(0.,0.,-1.));
#7237=DIRECTION('ref_axis',(1.,0.,0.));
#7238=DIRECTION('',(0.,0.,-1.));
#7239=DIRECTION('center_axis',(0.,0.,1.));
#7240=DIRECTION('ref_axis',(1.,0.,0.));
#7241=DIRECTION('center_axis',(0.,0.,-1.));
#7242=DIRECTION('ref_axis',(1.,0.,0.));
#7243=DIRECTION('center_axis',(0.,0.,-1.));
#7244=DIRECTION('ref_axis',(1.,0.,0.));
#7245=DIRECTION('',(0.,0.,-1.));
#7246=DIRECTION('center_axis',(0.,0.,1.));
#7247=DIRECTION('ref_axis',(1.,0.,0.));
#7248=DIRECTION('center_axis',(0.,0.,-1.));
#7249=DIRECTION('ref_axis',(1.,0.,0.));
#7250=DIRECTION('center_axis',(0.,0.,-1.));
#7251=DIRECTION('ref_axis',(1.,0.,0.));
#7252=DIRECTION('',(0.,0.,-1.));
#7253=DIRECTION('center_axis',(0.,0.,1.));
#7254=DIRECTION('ref_axis',(1.,0.,0.));
#7255=DIRECTION('center_axis',(0.,-1.,0.));
#7256=DIRECTION('ref_axis',(-1.,0.,0.));
#7257=DIRECTION('',(-1.,0.,0.));
#7258=DIRECTION('',(0.,0.,-1.));
#7259=DIRECTION('',(1.,0.,0.));
#7260=DIRECTION('',(0.,0.,-1.));
#7261=DIRECTION('center_axis',(1.,0.,0.));
#7262=DIRECTION('ref_axis',(0.,-1.,0.));
#7263=DIRECTION('',(0.,-1.,0.));
#7264=DIRECTION('',(0.,0.,-1.));
#7265=DIRECTION('',(0.,1.,0.));
#7266=DIRECTION('center_axis',(0.,1.,0.));
#7267=DIRECTION('ref_axis',(1.,0.,0.));
#7268=DIRECTION('',(1.,0.,0.));
#7269=DIRECTION('',(0.,0.,-1.));
#7270=DIRECTION('',(-1.,0.,0.));
#7271=DIRECTION('center_axis',(-1.,0.,0.));
#7272=DIRECTION('ref_axis',(0.,1.,0.));
#7273=DIRECTION('',(0.,1.,0.));
#7274=DIRECTION('',(0.,-1.,0.));
#7275=DIRECTION('center_axis',(0.,-1.,0.));
#7276=DIRECTION('ref_axis',(-1.,0.,0.));
#7277=DIRECTION('',(-1.,0.,0.));
#7278=DIRECTION('',(0.,0.,-1.));
#7279=DIRECTION('',(1.,0.,0.));
#7280=DIRECTION('',(0.,0.,-1.));
#7281=DIRECTION('center_axis',(1.,0.,0.));
#7282=DIRECTION('ref_axis',(0.,-1.,0.));
#7283=DIRECTION('',(0.,-1.,0.));
#7284=DIRECTION('',(0.,0.,-1.));
#7285=DIRECTION('',(0.,1.,0.));
#7286=DIRECTION('center_axis',(0.,1.,0.));
#7287=DIRECTION('ref_axis',(1.,0.,0.));
#7288=DIRECTION('',(1.,0.,0.));
#7289=DIRECTION('',(0.,0.,-1.));
#7290=DIRECTION('',(-1.,0.,0.));
#7291=DIRECTION('center_axis',(-1.,0.,0.));
#7292=DIRECTION('ref_axis',(0.,1.,0.));
#7293=DIRECTION('',(0.,1.,0.));
#7294=DIRECTION('',(0.,-1.,0.));
#7295=DIRECTION('center_axis',(0.,1.,0.));
#7296=DIRECTION('ref_axis',(-1.,0.,0.));
#7297=DIRECTION('',(1.,0.,0.));
#7298=DIRECTION('',(0.,0.,-1.));
#7299=DIRECTION('',(-1.,0.,0.));
#7300=DIRECTION('',(0.,0.,1.));
#7301=DIRECTION('center_axis',(0.,-1.,0.));
#7302=DIRECTION('ref_axis',(1.,0.,0.));
#7303=DIRECTION('',(-1.,0.,0.));
#7304=DIRECTION('',(0.,0.,1.));
#7305=DIRECTION('',(1.,0.,0.));
#7306=DIRECTION('',(0.,0.,1.));
#7307=DIRECTION('center_axis',(0.,0.,1.));
#7308=DIRECTION('ref_axis',(1.,0.,0.));
#7309=DIRECTION('',(0.,1.,0.));
#7310=DIRECTION('',(0.,1.,0.));
#7311=DIRECTION('center_axis',(0.,0.,1.));
#7312=DIRECTION('ref_axis',(1.,0.,0.));
#7313=DIRECTION('',(0.,1.,0.));
#7314=DIRECTION('',(1.,0.,0.));
#7315=DIRECTION('',(0.,1.,0.));
#7316=DIRECTION('center_axis',(0.,0.,1.));
#7317=DIRECTION('ref_axis',(1.,0.,0.));
#7318=DIRECTION('',(0.,1.,0.));
#7319=DIRECTION('',(1.,0.,0.));
#7320=DIRECTION('',(0.,1.,0.));
#7321=DIRECTION('center_axis',(0.,1.,0.));
#7322=DIRECTION('ref_axis',(-1.,0.,0.));
#7323=DIRECTION('',(0.,0.,-1.));
#7324=DIRECTION('',(-1.,0.,0.));
#7325=DIRECTION('',(0.,0.,1.));
#7326=DIRECTION('center_axis',(0.,-1.,0.));
#7327=DIRECTION('ref_axis',(1.,0.,0.));
#7328=DIRECTION('',(-1.,0.,0.));
#7329=DIRECTION('',(0.,0.,1.));
#7330=DIRECTION('',(1.,0.,0.));
#7331=DIRECTION('',(0.,0.,1.));
#7332=DIRECTION('center_axis',(0.,0.,1.));
#7333=DIRECTION('ref_axis',(1.,0.,0.));
#7334=DIRECTION('',(0.,1.,0.));
#7335=DIRECTION('',(0.,1.,0.));
#7336=DIRECTION('center_axis',(0.,0.,1.));
#7337=DIRECTION('ref_axis',(1.,0.,0.));
#7338=DIRECTION('',(0.,1.,0.));
#7339=DIRECTION('',(-1.,0.,0.));
#7340=DIRECTION('',(0.,1.,0.));
#7341=DIRECTION('center_axis',(0.,1.,0.));
#7342=DIRECTION('ref_axis',(-1.,0.,0.));
#7343=DIRECTION('',(1.,0.,0.));
#7344=DIRECTION('',(0.,0.,-1.));
#7345=DIRECTION('',(0.,0.,-1.));
#7346=DIRECTION('center_axis',(1.,0.,0.));
#7347=DIRECTION('ref_axis',(0.,1.,0.));
#7348=DIRECTION('',(0.,1.,0.));
#7349=DIRECTION('',(0.,0.,1.));
#7350=DIRECTION('center_axis',(0.,-1.,0.));
#7351=DIRECTION('ref_axis',(1.,0.,0.));
#7352=DIRECTION('',(-1.,0.,0.));
#7353=DIRECTION('',(0.,0.,1.));
#7354=DIRECTION('center_axis',(-1.,0.,0.));
#7355=DIRECTION('ref_axis',(0.,-1.,0.));
#7356=DIRECTION('',(0.,1.,0.));
#7357=DIRECTION('center_axis',(0.,0.,1.));
#7358=DIRECTION('ref_axis',(1.,0.,0.));
#8733=CARTESIAN_POINT('',(0.,0.,0.));
#8734=CARTESIAN_POINT('Origin',(83.,-23.,-4.));
#8735=CARTESIAN_POINT('',(79.5,-23.,-4.));
#8736=CARTESIAN_POINT('Origin',(83.,-23.,-4.));
#8737=CARTESIAN_POINT('',(80.5,-23.,-4.));
#8738=CARTESIAN_POINT('Origin',(83.,-23.,-4.));
#8739=CARTESIAN_POINT('Origin',(83.,-23.,-2.));
#8740=CARTESIAN_POINT('',(79.5,-23.,0.));
#8741=CARTESIAN_POINT('Origin',(83.,-23.,0.));
#8742=CARTESIAN_POINT('',(79.5,-23.,-2.));
#8743=CARTESIAN_POINT('Origin',(83.,-23.,-3.));
#8744=CARTESIAN_POINT('',(80.5,-23.,-6.));
#8745=CARTESIAN_POINT('',(80.5,-23.,-3.));
#8746=CARTESIAN_POINT('Origin',(83.,-23.,-6.));
#8747=CARTESIAN_POINT('Origin',(83.,23.,-4.));
#8748=CARTESIAN_POINT('',(79.5,23.,-4.));
#8749=CARTESIAN_POINT('Origin',(83.,23.,-4.));
#8750=CARTESIAN_POINT('',(80.5,23.,-4.));
#8751=CARTESIAN_POINT('Origin',(83.,23.,-4.));
#8752=CARTESIAN_POINT('Origin',(83.,23.,-2.));
#8753=CARTESIAN_POINT('',(79.5,23.,0.));
#8754=CARTESIAN_POINT('Origin',(83.,23.,0.));
#8755=CARTESIAN_POINT('',(79.5,23.,-2.));
#8756=CARTESIAN_POINT('Origin',(83.,23.,-3.));
#8757=CARTESIAN_POINT('',(80.5,23.,-6.));
#8758=CARTESIAN_POINT('',(80.5,23.,-3.));
#8759=CARTESIAN_POINT('Origin',(83.,23.,-6.));
#8760=CARTESIAN_POINT('Origin',(105.,-23.,-3.));
#8761=CARTESIAN_POINT('',(101.5,-23.,0.));
#8762=CARTESIAN_POINT('Origin',(105.,-23.,0.));
#8763=CARTESIAN_POINT('',(101.5,-23.,-6.));
#8764=CARTESIAN_POINT('',(101.5,-23.,-3.));
#8765=CARTESIAN_POINT('Origin',(105.,-23.,-6.));
#8766=CARTESIAN_POINT('Origin',(-105.,-23.,-3.));
#8767=CARTESIAN_POINT('',(-108.5,-23.,0.));
#8768=CARTESIAN_POINT('Origin',(-105.,-23.,0.));
#8769=CARTESIAN_POINT('',(-108.5,-23.,-6.));
#8770=CARTESIAN_POINT('',(-108.5,-23.,-3.));
#8771=CARTESIAN_POINT('Origin',(-105.,-23.,-6.));
#8772=CARTESIAN_POINT('Origin',(-105.,23.,-3.));
#8773=CARTESIAN_POINT('',(-108.5,23.,0.));
#8774=CARTESIAN_POINT('Origin',(-105.,23.,0.));
#8775=CARTESIAN_POINT('',(-108.5,23.,-6.));
#8776=CARTESIAN_POINT('',(-108.5,23.,-3.));
#8777=CARTESIAN_POINT('Origin',(-105.,23.,-6.));
#8778=CARTESIAN_POINT('Origin',(105.,23.,-3.));
#8779=CARTESIAN_POINT('',(101.5,23.,0.));
#8780=CARTESIAN_POINT('Origin',(105.,23.,0.));
#8781=CARTESIAN_POINT('',(101.5,23.,-6.));
#8782=CARTESIAN_POINT('',(101.5,23.,-3.));
#8783=CARTESIAN_POINT('Origin',(105.,23.,-6.));
#8784=CARTESIAN_POINT('Origin',(72.,-6.,0.));
#8785=CARTESIAN_POINT('',(72.,-6.,0.));
#8786=CARTESIAN_POINT('',(64.,-6.,0.));
#8787=CARTESIAN_POINT('',(36.,-6.,0.));
#8788=CARTESIAN_POINT('',(72.,-6.,-6.));
#8789=CARTESIAN_POINT('',(72.,-6.,0.));
#8790=CARTESIAN_POINT('',(64.,-6.,-6.));
#8791=CARTESIAN_POINT('',(36.,-6.,-6.));
#8792=CARTESIAN_POINT('',(64.,-6.,0.));
#8793=CARTESIAN_POINT('Origin',(72.,6.,0.));
#8794=CARTESIAN_POINT('',(72.,6.,0.));
#8795=CARTESIAN_POINT('',(72.,3.,0.));
#8796=CARTESIAN_POINT('',(72.,6.,-6.));
#8797=CARTESIAN_POINT('',(72.,6.,0.));
#8798=CARTESIAN_POINT('',(72.,3.,-6.));
#8799=CARTESIAN_POINT('Origin',(64.,6.,0.));
#8800=CARTESIAN_POINT('',(64.,6.,0.));
#8801=CARTESIAN_POINT('',(32.,6.,0.));
#8802=CARTESIAN_POINT('',(64.,6.,-6.));
#8803=CARTESIAN_POINT('',(64.,6.,0.));
#8804=CARTESIAN_POINT('',(32.,6.,-6.));
#8805=CARTESIAN_POINT('Origin',(64.,-6.,0.));
#8806=CARTESIAN_POINT('',(64.,-3.,0.));
#8807=CARTESIAN_POINT('',(64.,-3.,-6.));
#8808=CARTESIAN_POINT('Origin',(102.,-6.,0.));
#8809=CARTESIAN_POINT('',(102.,-6.,0.));
#8810=CARTESIAN_POINT('',(94.,-6.,0.));
#8811=CARTESIAN_POINT('',(51.,-6.,0.));
#8812=CARTESIAN_POINT('',(102.,-6.,-6.));
#8813=CARTESIAN_POINT('',(102.,-6.,0.));
#8814=CARTESIAN_POINT('',(94.,-6.,-6.));
#8815=CARTESIAN_POINT('',(51.,-6.,-6.));
#8816=CARTESIAN_POINT('',(94.,-6.,0.));
#8817=CARTESIAN_POINT('Origin',(102.,6.,0.));
#8818=CARTESIAN_POINT('',(102.,6.,0.));
#8819=CARTESIAN_POINT('',(102.,3.,0.));
#8820=CARTESIAN_POINT('',(102.,6.,-6.));
#8821=CARTESIAN_POINT('',(102.,6.,0.));
#8822=CARTESIAN_POINT('',(102.,3.,-6.));
#8823=CARTESIAN_POINT('Origin',(94.,6.,0.));
#8824=CARTESIAN_POINT('',(94.,6.,0.));
#8825=CARTESIAN_POINT('',(47.,6.,0.));
#8826=CARTESIAN_POINT('',(94.,6.,-6.));
#8827=CARTESIAN_POINT('',(94.,6.,0.));
#8828=CARTESIAN_POINT('',(47.,6.,-6.));
#8829=CARTESIAN_POINT('Origin',(94.,-6.,0.));
#8830=CARTESIAN_POINT('',(94.,-3.,0.));
#8831=CARTESIAN_POINT('',(94.,-3.,-6.));
#8832=CARTESIAN_POINT('Origin',(120.,15.,0.));
#8833=CARTESIAN_POINT('',(-125.,15.,0.));
#8834=CARTESIAN_POINT('',(120.,15.,0.));
#8835=CARTESIAN_POINT('',(60.,15.,0.));
#8836=CARTESIAN_POINT('',(-125.,15.,25.));
#8837=CARTESIAN_POINT('',(-125.,15.,-3.));
#8838=CARTESIAN_POINT('',(120.,15.,25.));
#8839=CARTESIAN_POINT('',(120.,15.,25.));
#8840=CARTESIAN_POINT('',(120.,15.,0.));
#8841=CARTESIAN_POINT('Origin',(-120.,11.,0.));
#8842=CARTESIAN_POINT('',(120.,11.,0.));
#8843=CARTESIAN_POINT('',(-125.,11.,0.));
#8844=CARTESIAN_POINT('',(-60.,11.,0.));
#8845=CARTESIAN_POINT('',(120.,11.,25.));
#8846=CARTESIAN_POINT('',(120.,11.,0.));
#8847=CARTESIAN_POINT('',(-125.,11.,25.));
#8848=CARTESIAN_POINT('',(-120.,11.,25.));
#8849=CARTESIAN_POINT('',(-125.,11.,-3.));
#8850=CARTESIAN_POINT('Origin',(0.,13.,25.));
#8851=CARTESIAN_POINT('',(-125.,21.5,25.));
#8852=CARTESIAN_POINT('',(120.,11.,25.));
#8853=CARTESIAN_POINT('Origin',(0.,0.,0.));
#8854=CARTESIAN_POINT('',(120.,35.,0.));
#8855=CARTESIAN_POINT('',(120.,-30.,0.));
#8856=CARTESIAN_POINT('',(-125.,35.,0.));
#8857=CARTESIAN_POINT('',(60.,35.,0.));
#8858=CARTESIAN_POINT('',(-125.,15.,0.));
#8859=CARTESIAN_POINT('Origin',(0.,0.,0.));
#8860=CARTESIAN_POINT('',(-125.,-11.,0.));
#8861=CARTESIAN_POINT('',(-125.,15.,0.));
#8862=CARTESIAN_POINT('',(120.,-11.,0.));
#8863=CARTESIAN_POINT('',(60.,-11.,0.));
#8864=CARTESIAN_POINT('',(120.,-30.,0.));
#8865=CARTESIAN_POINT('Origin',(120.,-11.,0.));
#8866=CARTESIAN_POINT('',(-125.,-11.,22.));
#8867=CARTESIAN_POINT('',(-125.,-11.,-3.));
#8868=CARTESIAN_POINT('',(120.,-11.,22.));
#8869=CARTESIAN_POINT('',(120.,-11.,22.));
#8870=CARTESIAN_POINT('',(120.,-11.,0.));
#8871=CARTESIAN_POINT('Origin',(-120.,-15.,0.));
#8872=CARTESIAN_POINT('',(120.,-15.,0.));
#8873=CARTESIAN_POINT('',(-125.,-15.,0.));
#8874=CARTESIAN_POINT('',(-60.,-15.,0.));
#8875=CARTESIAN_POINT('',(120.,-15.,22.));
#8876=CARTESIAN_POINT('',(120.,-15.,0.));
#8877=CARTESIAN_POINT('',(-125.,-15.,22.));
#8878=CARTESIAN_POINT('',(-120.,-15.,22.));
#8879=CARTESIAN_POINT('',(-125.,-15.,-3.));
#8880=CARTESIAN_POINT('Origin',(0.,-13.,22.));
#8881=CARTESIAN_POINT('',(-125.,8.5,22.));
#8882=CARTESIAN_POINT('',(120.,-15.,22.));
#8883=CARTESIAN_POINT('Origin',(0.,0.,0.));
#8884=CARTESIAN_POINT('',(-125.,-35.,0.));
#8885=CARTESIAN_POINT('',(-125.,15.,0.));
#8886=CARTESIAN_POINT('',(120.,-35.,0.));
#8887=CARTESIAN_POINT('',(-60.,-35.,0.));
#8888=CARTESIAN_POINT('',(120.,-30.,0.));
#8889=CARTESIAN_POINT('Origin',(120.,35.,-6.));
#8890=CARTESIAN_POINT('',(120.,35.,-6.));
#8891=CARTESIAN_POINT('',(-125.,35.,-6.));
#8892=CARTESIAN_POINT('',(60.,35.,-6.));
#8893=CARTESIAN_POINT('',(-125.,35.,-6.));
#8894=CARTESIAN_POINT('',(120.,35.,-6.));
#8895=CARTESIAN_POINT('Origin',(120.,-30.,-6.));
#8896=CARTESIAN_POINT('',(120.,-35.,-6.));
#8897=CARTESIAN_POINT('',(120.,-30.,-6.));
#8898=CARTESIAN_POINT('',(120.,-35.,-6.));
#8899=CARTESIAN_POINT('Origin',(-120.,-35.,-6.));
#8900=CARTESIAN_POINT('',(-125.,-35.,-6.));
#8901=CARTESIAN_POINT('',(-60.,-35.,-6.));
#8902=CARTESIAN_POINT('',(-125.,-35.,-6.));
#8903=CARTESIAN_POINT('Origin',(-125.,30.,-6.));
#8904=CARTESIAN_POINT('',(-125.,15.,-6.));
#8905=CARTESIAN_POINT('Origin',(0.,0.,-6.));
#19823=UNCERTAINTY_MEASURE_WITH_UNIT(LENGTH_MEASURE(0.01),#19864,
'DISTANCE_ACCURACY_VALUE',
'Maximum model space distance between geometric entities at asserted c
onnectivities');
#19842=UNCERTAINTY_MEASURE_WITH_UNIT(LENGTH_MEASURE(0.01),#19864,
'DISTANCE_ACCURACY_VALUE',
'Maximum model space distance between geometric entities at asserted c
onnectivities');
#19844=(
GEOMETRIC_REPRESENTATION_CONTEXT(3)
GLOBAL_UNCERTAINTY_ASSIGNED_CONTEXT((#19823))
GLOBAL_UNIT_ASSIGNED_CONTEXT((#19864,#19866,#19867))
REPRESENTATION_CONTEXT('','3D')
);
#19863=(
GEOMETRIC_REPRESENTATION_CONTEXT(3)
GLOBAL_UNCERTAINTY_ASSIGNED_CONTEXT((#19842))
GLOBAL_UNIT_ASSIGNED_CONTEXT((#19864,#19866,#19867))
REPRESENTATION_CONTEXT('','3D')
);
#19864=(
LENGTH_UNIT()
NAMED_UNIT(*)
SI_UNIT(.MILLI.,.METRE.)
);
#19866=(
NAMED_UNIT(*)
PLANE_ANGLE_UNIT()
SI_UNIT($,.RADIAN.)
);
#19867=(
NAMED_UNIT(*)
SI_UNIT($,.STERADIAN.)
SOLID_ANGLE_UNIT()
);
#19869=SHAPE_DEFINITION_REPRESENTATION(#19889,#19935);
#19889=PRODUCT_DEFINITION_SHAPE('',$,#19956);
#19935=SHAPE_REPRESENTATION('',(#6654),#19844);
#19954=PRODUCT_DEFINITION_CONTEXT('part definition',#20016,'design');
#19956=PRODUCT_DEFINITION('Track channel','Track channel',#19976,#19954);
#19976=PRODUCT_DEFINITION_FORMATION('',$,#20019);
#20016=APPLICATION_CONTEXT(
'Core Data for Automotive Mechanical Design Process');
#20017=PRODUCT_CONTEXT('part definition',#20016,'mechanical');
#20019=PRODUCT('Track channel','Track channel',$,(#20017));
#20039=PRESENTATION_STYLE_ASSIGNMENT((#20046));
#20046=SURFACE_STYLE_USAGE(.BOTH.,#20053);
#20053=SURFACE_SIDE_STYLE('',(#20060));
#20060=SURFACE_STYLE_FILL_AREA(#20067);
#20067=FILL_AREA_STYLE('Dark blue',(#20074));
#20074=FILL_AREA_STYLE_COLOUR('Dark blue',#20081);
#20081=COLOUR_RGB('Dark blue',0.0901960784313725,0.270588235294118,0.513725490196078);
ENDSEC;
END-ISO-10303-21;
